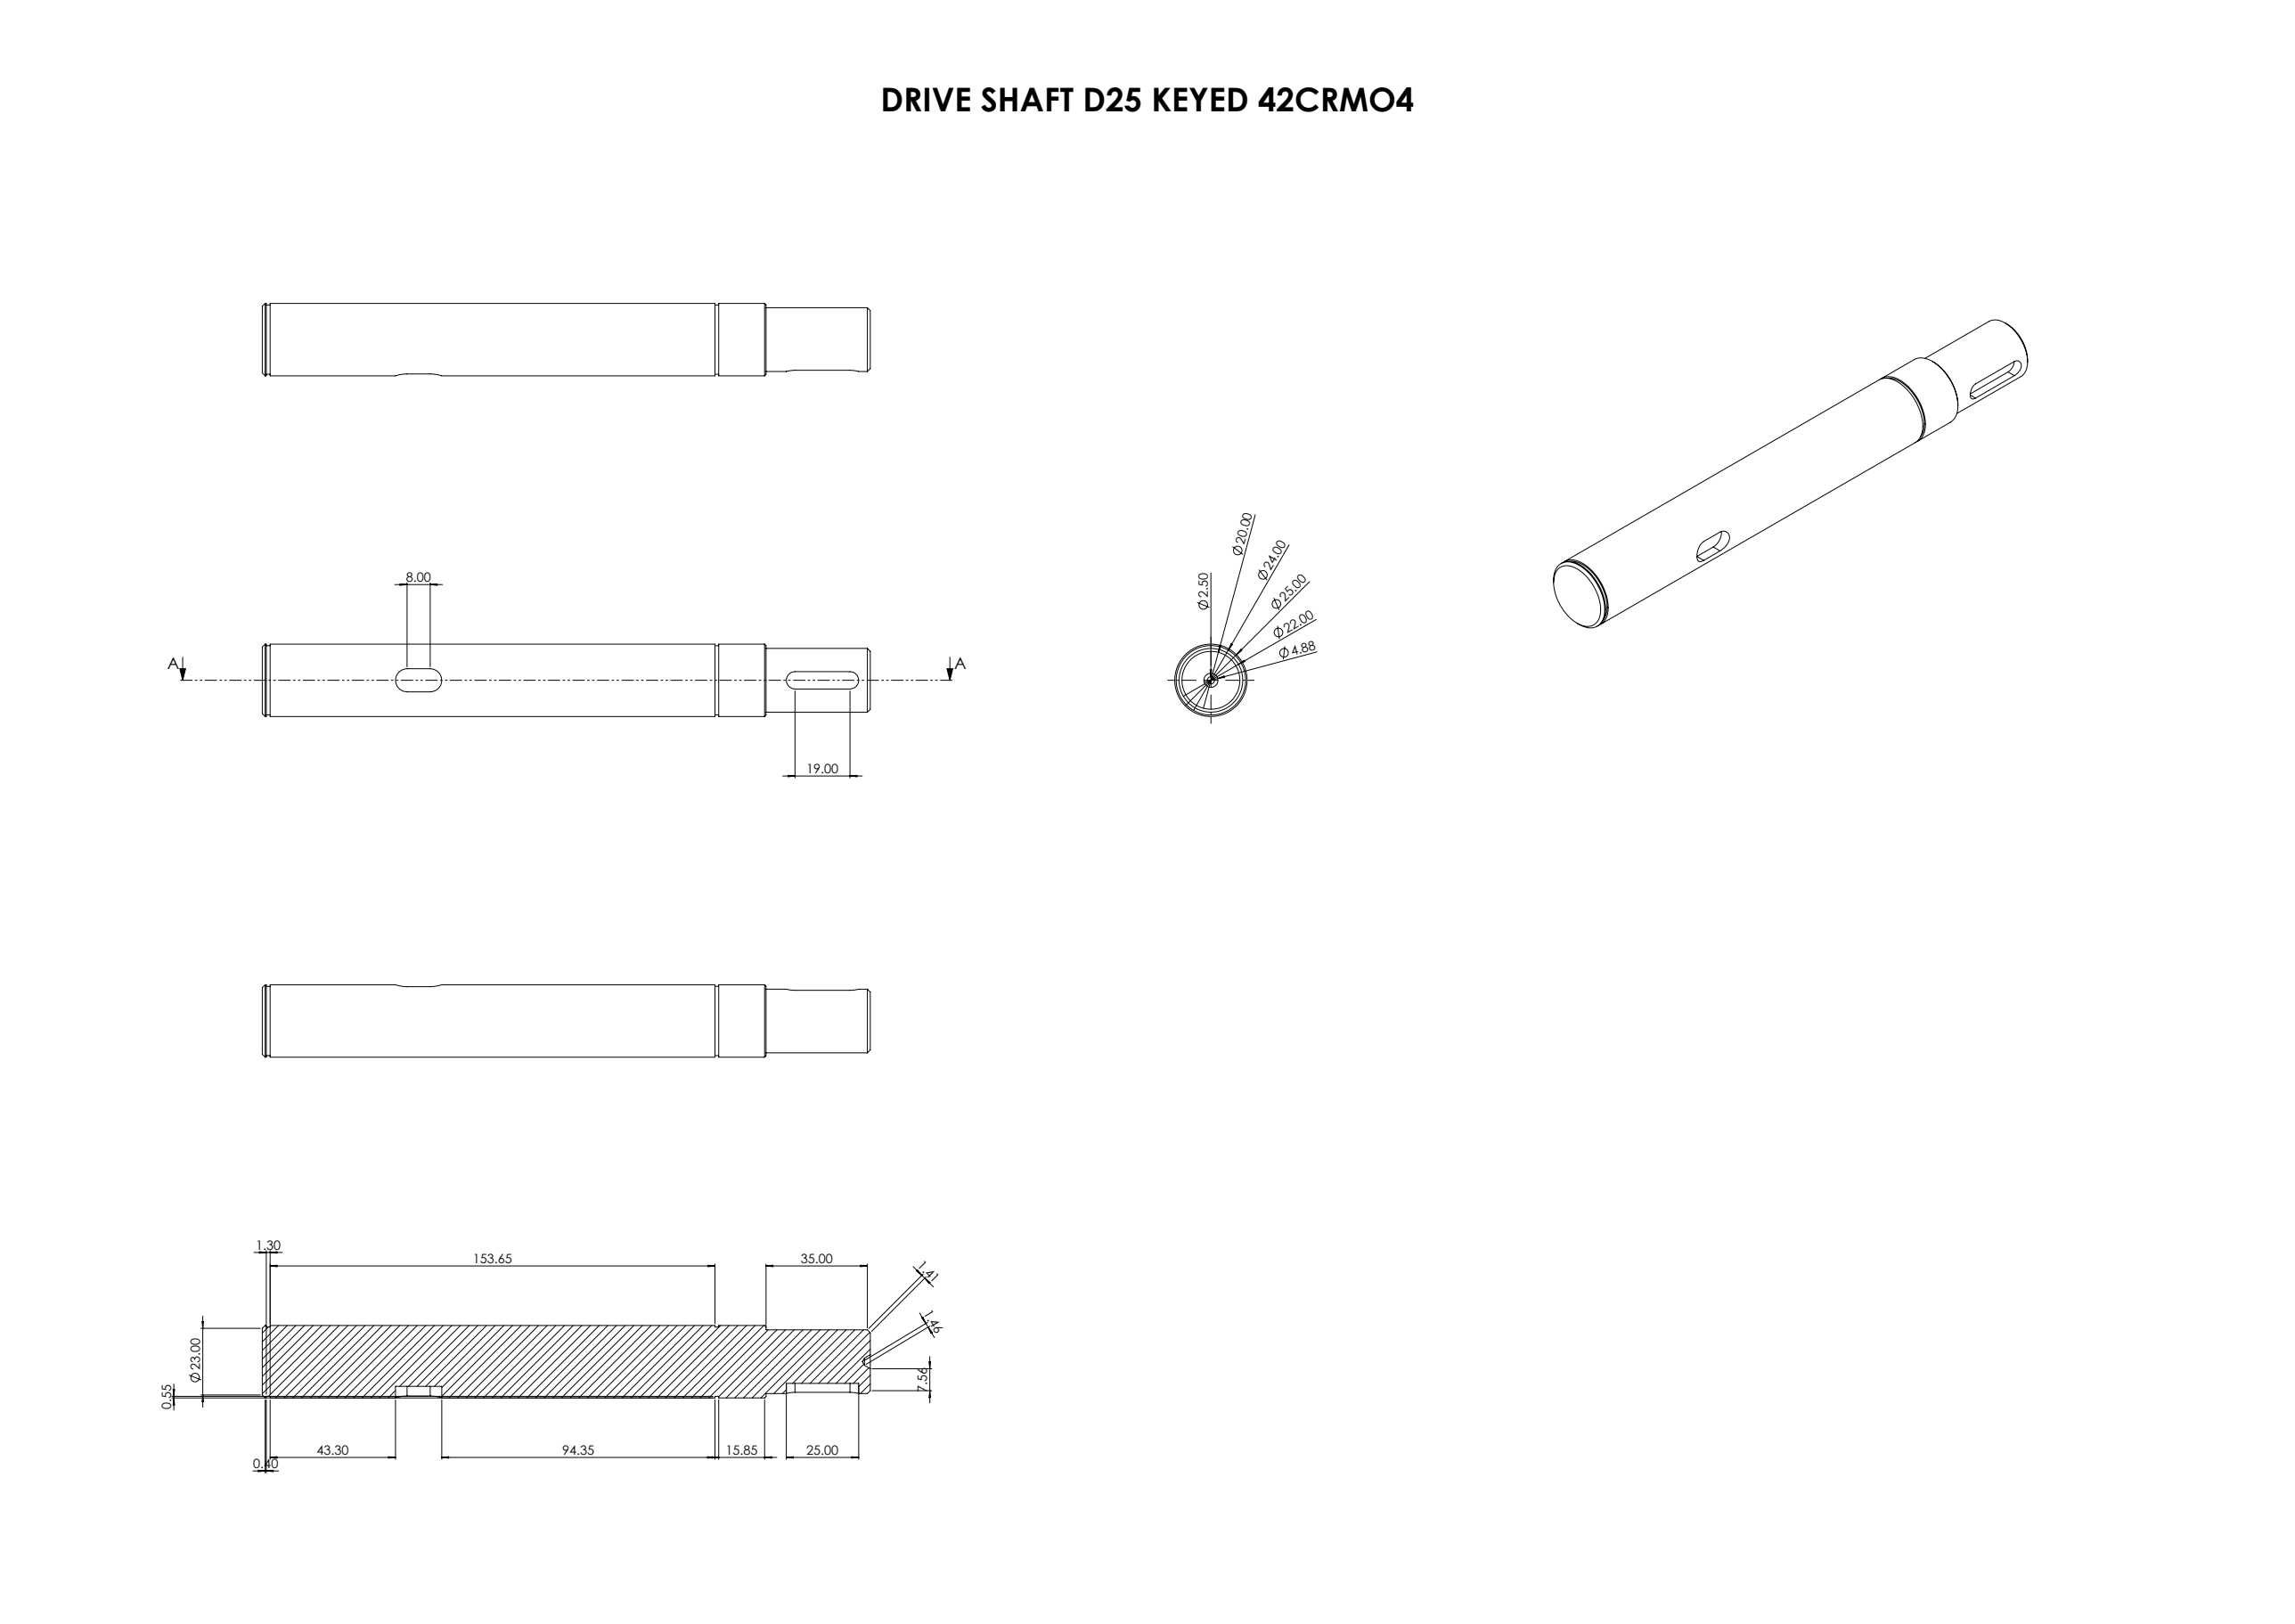
ISO-10303-21;
HEADER;
/* Generated by software containing ST-Developer
 * from STEP Tools, Inc. (www.steptools.com) 
 */

FILE_DESCRIPTION(
/* description */ (''),
/* implementation_level */ '2;1');

FILE_NAME(
/* name */ '04_Drive_Shaft_D25_Keyed_42CrMo4.step',
/* time_stamp */ '2026-10-23T00:52:27+05:00',
/* author */ (''),
/* organization */ (''),
/* preprocessor_version */ 'ST-DEVELOPER v20.2',
/* originating_system */ 'Autodesk Translation Framework v15.15.0.0',
/* authorisation */ '');

FILE_SCHEMA (('AUTOMOTIVE_DESIGN { 1 0 10303 214 3 1 1 }'));
ENDSEC;

DATA;
#10=MECHANICAL_DESIGN_GEOMETRIC_PRESENTATION_REPRESENTATION('',(#1556),#59204);
#679=B_SPLINE_CURVE_WITH_KNOTS('',3,(#41868,#41869,#41870,#41871,#41872,
#41873,#41874,#41875,#41876,#41877,#41878,#41879,#41880,#41881,#41882,#41883,
#41884,#41885),.UNSPECIFIED.,.F.,.F.,(4,2,2,2,2,2,2,2,4),(-0.909033920514541,
-0.795393296746547,-0.681752672978553,-0.568134816617911,-0.45451696025727,
-0.340899103896629,-0.227281247535988,-0.113640623767994,0.),
 .UNSPECIFIED.);
#680=B_SPLINE_CURVE_WITH_KNOTS('',3,(#41896,#41897,#41898,#41899,#41900,
#41901,#41902,#41903,#41904,#41905,#41906,#41907,#41908,#41909,#41910,#41911,
#41912,#41913),.UNSPECIFIED.,.F.,.F.,(4,2,2,2,2,2,2,2,4),(0.,0.113640623767995,
0.22728124753599,0.34089910389663,0.454516960257271,0.568134816617911,0.681752672978552,
0.795393296746547,0.909033920514541),.UNSPECIFIED.);
#681=B_SPLINE_CURVE_WITH_KNOTS('',3,(#41927,#41928,#41929,#41930,#41931,
#41932,#41933,#41934,#41935,#41936,#41937,#41938,#41939,#41940,#41941,#41942,
#41943,#41944),.UNSPECIFIED.,.F.,.F.,(4,2,2,2,2,2,2,2,4),(-1.21468374386295,
-1.06281862619298,-0.910953508522999,-0.759147690227238,-0.607341871931477,
-0.455536053635716,-0.303730235339955,-0.151865117669978,0.),
 .UNSPECIFIED.);
#682=B_SPLINE_CURVE_WITH_KNOTS('',3,(#41955,#41956,#41957,#41958,#41959,
#41960,#41961,#41962,#41963,#41964,#41965,#41966,#41967,#41968,#41969,#41970,
#41971,#41972),.UNSPECIFIED.,.F.,.F.,(4,2,2,2,2,2,2,2,4),(0.,0.151865117669977,
0.303730235339955,0.455536053635716,0.607341871931477,0.759147690227237,
0.910953508522998,1.06281862619298,1.21468374386295),.UNSPECIFIED.);
#1516=SHAPE_REPRESENTATION_RELATIONSHIP('SRR','None',#59305,#1536);
#1536=ADVANCED_BREP_SHAPE_REPRESENTATION('',(#1583),#59192);
#1556=STYLED_ITEM('',(#59586),#1583);
#1583=MANIFOLD_SOLID_BREP('Drive shaft',#22812);
#1639=FACE_BOUND('',#4332,.T.);
#1640=FACE_BOUND('',#4335,.T.);
#1641=FACE_BOUND('',#4337,.T.);
#1642=FACE_BOUND('',#4341,.T.);
#1643=FACE_BOUND('',#4344,.T.);
#1644=FACE_BOUND('',#4346,.T.);
#1645=FACE_BOUND('',#4348,.T.);
#1646=FACE_BOUND('',#4351,.T.);
#1990=PLANE('',#23564);
#1991=PLANE('',#23567);
#1992=PLANE('',#23570);
#1993=PLANE('',#23571);
#1994=PLANE('',#23574);
#1995=PLANE('',#23577);
#1996=PLANE('',#23578);
#1997=PLANE('',#23584);
#1998=PLANE('',#23590);
#1999=PLANE('',#23594);
#2000=PLANE('',#23598);
#2001=PLANE('',#23602);
#2002=PLANE('',#23608);
#2471=CYLINDRICAL_SURFACE('',#23565,0.3);
#2472=CYLINDRICAL_SURFACE('',#23568,0.3);
#2473=CYLINDRICAL_SURFACE('',#23572,0.4);
#2474=CYLINDRICAL_SURFACE('',#23575,0.4);
#2475=CYLINDRICAL_SURFACE('',#23582,1.1);
#2476=CYLINDRICAL_SURFACE('',#23588,1.25);
#2477=CYLINDRICAL_SURFACE('',#23592,1.195);
#2478=CYLINDRICAL_SURFACE('',#23596,1.25);
#2479=CYLINDRICAL_SURFACE('',#23600,1.195);
#2480=CYLINDRICAL_SURFACE('',#23604,1.25);
#2974=FACE_OUTER_BOUND('',#4319,.T.);
#2975=FACE_OUTER_BOUND('',#4320,.T.);
#2976=FACE_OUTER_BOUND('',#4321,.T.);
#2977=FACE_OUTER_BOUND('',#4322,.T.);
#2978=FACE_OUTER_BOUND('',#4323,.T.);
#2979=FACE_OUTER_BOUND('',#4324,.T.);
#2980=FACE_OUTER_BOUND('',#4325,.T.);
#2981=FACE_OUTER_BOUND('',#4326,.T.);
#2982=FACE_OUTER_BOUND('',#4327,.T.);
#2983=FACE_OUTER_BOUND('',#4328,.T.);
#2984=FACE_OUTER_BOUND('',#4329,.T.);
#2985=FACE_OUTER_BOUND('',#4330,.T.);
#2986=FACE_OUTER_BOUND('',#4331,.T.);
#2987=FACE_OUTER_BOUND('',#4333,.T.);
#2988=FACE_OUTER_BOUND('',#4334,.T.);
#2989=FACE_OUTER_BOUND('',#4336,.T.);
#2990=FACE_OUTER_BOUND('',#4338,.T.);
#2991=FACE_OUTER_BOUND('',#4339,.T.);
#2992=FACE_OUTER_BOUND('',#4340,.T.);
#2993=FACE_OUTER_BOUND('',#4342,.T.);
#2994=FACE_OUTER_BOUND('',#4343,.T.);
#2995=FACE_OUTER_BOUND('',#4345,.T.);
#2996=FACE_OUTER_BOUND('',#4347,.T.);
#2997=FACE_OUTER_BOUND('',#4349,.T.);
#2998=FACE_OUTER_BOUND('',#4350,.T.);
#2999=FACE_OUTER_BOUND('',#4352,.T.);
#3000=FACE_OUTER_BOUND('',#4353,.T.);
#3001=FACE_OUTER_BOUND('',#4354,.T.);
#4319=EDGE_LOOP('',(#16112,#16113,#16114,#16115));
#4320=EDGE_LOOP('',(#16116,#16117,#16118));
#4321=EDGE_LOOP('',(#16119,#16120,#16121,#16122));
#4322=EDGE_LOOP('',(#16123,#16124,#16125,#16126));
#4323=EDGE_LOOP('',(#16127,#16128,#16129,#16130));
#4324=EDGE_LOOP('',(#16131,#16132,#16133,#16134));
#4325=EDGE_LOOP('',(#16135,#16136,#16137,#16138));
#4326=EDGE_LOOP('',(#16139,#16140,#16141,#16142));
#4327=EDGE_LOOP('',(#16143,#16144,#16145,#16146));
#4328=EDGE_LOOP('',(#16147,#16148,#16149,#16150));
#4329=EDGE_LOOP('',(#16151,#16152,#16153,#16154));
#4330=EDGE_LOOP('',(#16155,#16156,#16157,#16158));
#4331=EDGE_LOOP('',(#16159));
#4332=EDGE_LOOP('',(#16160));
#4333=EDGE_LOOP('',(#16161,#16162,#16163,#16164));
#4334=EDGE_LOOP('',(#16165,#16166,#16167,#16168));
#4335=EDGE_LOOP('',(#16169,#16170,#16171,#16172));
#4336=EDGE_LOOP('',(#16173));
#4337=EDGE_LOOP('',(#16174));
#4338=EDGE_LOOP('',(#16175,#16176,#16177,#16178));
#4339=EDGE_LOOP('',(#16179,#16180,#16181,#16182));
#4340=EDGE_LOOP('',(#16183));
#4341=EDGE_LOOP('',(#16184));
#4342=EDGE_LOOP('',(#16185,#16186,#16187,#16188));
#4343=EDGE_LOOP('',(#16189));
#4344=EDGE_LOOP('',(#16190));
#4345=EDGE_LOOP('',(#16191,#16192,#16193,#16194));
#4346=EDGE_LOOP('',(#16195,#16196,#16197,#16198));
#4347=EDGE_LOOP('',(#16199));
#4348=EDGE_LOOP('',(#16200));
#4349=EDGE_LOOP('',(#16201,#16202,#16203,#16204));
#4350=EDGE_LOOP('',(#16205));
#4351=EDGE_LOOP('',(#16206));
#4352=EDGE_LOOP('',(#16207,#16208,#16209,#16210));
#4353=EDGE_LOOP('',(#16211,#16212,#16213,#16214));
#4354=EDGE_LOOP('',(#16215));
#5857=LINE('',#41852,#7290);
#5858=LINE('',#41856,#7291);
#5859=LINE('',#41860,#7292);
#5860=LINE('',#41862,#7293);
#5861=LINE('',#41864,#7294);
#5862=LINE('',#41865,#7295);
#5863=LINE('',#41888,#7296);
#5864=LINE('',#41891,#7297);
#5865=LINE('',#41893,#7298);
#5866=LINE('',#41894,#7299);
#5867=LINE('',#41919,#7300);
#5868=LINE('',#41921,#7301);
#5869=LINE('',#41923,#7302);
#5870=LINE('',#41924,#7303);
#5871=LINE('',#41947,#7304);
#5872=LINE('',#41950,#7305);
#5873=LINE('',#41952,#7306);
#5874=LINE('',#41953,#7307);
#5875=LINE('',#41981,#7308);
#5876=LINE('',#41985,#7309);
#5877=LINE('',#41992,#7310);
#5878=LINE('',#41996,#7311);
#5879=LINE('',#42003,#7312);
#5880=LINE('',#42010,#7313);
#5881=LINE('',#42017,#7314);
#5882=LINE('',#42024,#7315);
#5883=LINE('',#42028,#7316);
#7290=VECTOR('',#26517,0.1875);
#7291=VECTOR('',#26522,0.125);
#7292=VECTOR('',#26525,1.);
#7293=VECTOR('',#26526,1.);
#7294=VECTOR('',#26527,1.);
#7295=VECTOR('',#26528,1.);
#7296=VECTOR('',#26533,1.);
#7297=VECTOR('',#26536,1.);
#7298=VECTOR('',#26537,1.);
#7299=VECTOR('',#26538,1.);
#7300=VECTOR('',#26547,1.);
#7301=VECTOR('',#26548,1.);
#7302=VECTOR('',#26549,1.);
#7303=VECTOR('',#26550,1.);
#7304=VECTOR('',#26555,1.);
#7305=VECTOR('',#26558,1.);
#7306=VECTOR('',#26559,1.);
#7307=VECTOR('',#26560,1.);
#7308=VECTOR('',#26575,1.05);
#7309=VECTOR('',#26580,1.1);
#7310=VECTOR('',#26589,1.225);
#7311=VECTOR('',#26594,1.25);
#7312=VECTOR('',#26603,1.195);
#7313=VECTOR('',#26612,1.25);
#7314=VECTOR('',#26621,1.195);
#7315=VECTOR('',#26630,1.25);
#7316=VECTOR('',#26635,1.2);
#8574=CIRCLE('',#23561,0.24404761904762);
#8575=CIRCLE('',#23562,0.125);
#8576=CIRCLE('',#23566,0.3);
#8577=CIRCLE('',#23569,0.3);
#8578=CIRCLE('',#23573,0.4);
#8579=CIRCLE('',#23576,0.4);
#8580=CIRCLE('',#23579,1.);
#8581=CIRCLE('',#23581,1.1);
#8582=CIRCLE('',#23583,1.1);
#8583=CIRCLE('',#23585,1.2);
#8584=CIRCLE('',#23587,1.25);
#8585=CIRCLE('',#23589,1.25);
#8586=CIRCLE('',#23591,1.195);
#8587=CIRCLE('',#23593,1.195);
#8588=CIRCLE('',#23595,1.25);
#8589=CIRCLE('',#23597,1.25);
#8590=CIRCLE('',#23599,1.195);
#8591=CIRCLE('',#23601,1.195);
#8592=CIRCLE('',#23603,1.25);
#8593=CIRCLE('',#23605,1.25);
#8594=CIRCLE('',#23607,1.15);
#9642=VERTEX_POINT('',#41849);
#9643=VERTEX_POINT('',#41851);
#9644=VERTEX_POINT('',#41855);
#9645=VERTEX_POINT('',#41858);
#9646=VERTEX_POINT('',#41859);
#9647=VERTEX_POINT('',#41861);
#9648=VERTEX_POINT('',#41863);
#9649=VERTEX_POINT('',#41867);
#9650=VERTEX_POINT('',#41886);
#9651=VERTEX_POINT('',#41890);
#9652=VERTEX_POINT('',#41892);
#9653=VERTEX_POINT('',#41917);
#9654=VERTEX_POINT('',#41918);
#9655=VERTEX_POINT('',#41920);
#9656=VERTEX_POINT('',#41922);
#9657=VERTEX_POINT('',#41926);
#9658=VERTEX_POINT('',#41945);
#9659=VERTEX_POINT('',#41949);
#9660=VERTEX_POINT('',#41951);
#9661=VERTEX_POINT('',#41976);
#9662=VERTEX_POINT('',#41979);
#9663=VERTEX_POINT('',#41983);
#9664=VERTEX_POINT('',#41987);
#9665=VERTEX_POINT('',#41990);
#9666=VERTEX_POINT('',#41994);
#9667=VERTEX_POINT('',#41998);
#9668=VERTEX_POINT('',#42001);
#9669=VERTEX_POINT('',#42005);
#9670=VERTEX_POINT('',#42008);
#9671=VERTEX_POINT('',#42012);
#9672=VERTEX_POINT('',#42015);
#9673=VERTEX_POINT('',#42019);
#9674=VERTEX_POINT('',#42022);
#9675=VERTEX_POINT('',#42026);
#12060=EDGE_CURVE('',#9642,#9642,#8574,.T.);
#12061=EDGE_CURVE('',#9642,#9643,#5857,.T.);
#12062=EDGE_CURVE('',#9643,#9643,#8575,.T.);
#12063=EDGE_CURVE('',#9643,#9644,#5858,.T.);
#12064=EDGE_CURVE('',#9645,#9646,#5859,.T.);
#12065=EDGE_CURVE('',#9647,#9645,#5860,.T.);
#12066=EDGE_CURVE('',#9647,#9648,#5861,.T.);
#12067=EDGE_CURVE('',#9648,#9646,#5862,.T.);
#12068=EDGE_CURVE('',#9646,#9649,#679,.T.);
#12069=EDGE_CURVE('',#9650,#9648,#8576,.T.);
#12070=EDGE_CURVE('',#9650,#9649,#5863,.T.);
#12071=EDGE_CURVE('',#9649,#9651,#5864,.T.);
#12072=EDGE_CURVE('',#9650,#9652,#5865,.T.);
#12073=EDGE_CURVE('',#9652,#9651,#5866,.T.);
#12074=EDGE_CURVE('',#9651,#9645,#680,.T.);
#12075=EDGE_CURVE('',#9647,#9652,#8577,.T.);
#12076=EDGE_CURVE('',#9653,#9654,#5867,.T.);
#12077=EDGE_CURVE('',#9655,#9653,#5868,.T.);
#12078=EDGE_CURVE('',#9655,#9656,#5869,.T.);
#12079=EDGE_CURVE('',#9656,#9654,#5870,.T.);
#12080=EDGE_CURVE('',#9654,#9657,#681,.T.);
#12081=EDGE_CURVE('',#9658,#9656,#8578,.T.);
#12082=EDGE_CURVE('',#9658,#9657,#5871,.T.);
#12083=EDGE_CURVE('',#9657,#9659,#5872,.T.);
#12084=EDGE_CURVE('',#9658,#9660,#5873,.T.);
#12085=EDGE_CURVE('',#9660,#9659,#5874,.T.);
#12086=EDGE_CURVE('',#9659,#9653,#682,.T.);
#12087=EDGE_CURVE('',#9655,#9660,#8579,.T.);
#12088=EDGE_CURVE('',#9661,#9661,#8580,.T.);
#12089=EDGE_CURVE('',#9662,#9662,#8581,.T.);
#12090=EDGE_CURVE('',#9662,#9661,#5875,.T.);
#12091=EDGE_CURVE('',#9663,#9663,#8582,.T.);
#12092=EDGE_CURVE('',#9663,#9662,#5876,.T.);
#12093=EDGE_CURVE('',#9664,#9664,#8583,.T.);
#12094=EDGE_CURVE('',#9665,#9665,#8584,.T.);
#12095=EDGE_CURVE('',#9665,#9664,#5877,.T.);
#12096=EDGE_CURVE('',#9666,#9666,#8585,.T.);
#12097=EDGE_CURVE('',#9666,#9665,#5878,.T.);
#12098=EDGE_CURVE('',#9667,#9667,#8586,.T.);
#12099=EDGE_CURVE('',#9668,#9668,#8587,.T.);
#12100=EDGE_CURVE('',#9668,#9667,#5879,.T.);
#12101=EDGE_CURVE('',#9669,#9669,#8588,.T.);
#12102=EDGE_CURVE('',#9670,#9670,#8589,.T.);
#12103=EDGE_CURVE('',#9670,#9669,#5880,.T.);
#12104=EDGE_CURVE('',#9671,#9671,#8590,.T.);
#12105=EDGE_CURVE('',#9672,#9672,#8591,.T.);
#12106=EDGE_CURVE('',#9672,#9671,#5881,.T.);
#12107=EDGE_CURVE('',#9673,#9673,#8592,.T.);
#12108=EDGE_CURVE('',#9674,#9674,#8593,.T.);
#12109=EDGE_CURVE('',#9674,#9673,#5882,.T.);
#12110=EDGE_CURVE('',#9675,#9675,#8594,.T.);
#12111=EDGE_CURVE('',#9675,#9674,#5883,.T.);
#16112=ORIENTED_EDGE('',*,*,#12060,.F.);
#16113=ORIENTED_EDGE('',*,*,#12061,.T.);
#16114=ORIENTED_EDGE('',*,*,#12062,.T.);
#16115=ORIENTED_EDGE('',*,*,#12061,.F.);
#16116=ORIENTED_EDGE('',*,*,#12062,.F.);
#16117=ORIENTED_EDGE('',*,*,#12063,.T.);
#16118=ORIENTED_EDGE('',*,*,#12063,.F.);
#16119=ORIENTED_EDGE('',*,*,#12064,.F.);
#16120=ORIENTED_EDGE('',*,*,#12065,.F.);
#16121=ORIENTED_EDGE('',*,*,#12066,.T.);
#16122=ORIENTED_EDGE('',*,*,#12067,.T.);
#16123=ORIENTED_EDGE('',*,*,#12068,.F.);
#16124=ORIENTED_EDGE('',*,*,#12067,.F.);
#16125=ORIENTED_EDGE('',*,*,#12069,.F.);
#16126=ORIENTED_EDGE('',*,*,#12070,.T.);
#16127=ORIENTED_EDGE('',*,*,#12071,.F.);
#16128=ORIENTED_EDGE('',*,*,#12070,.F.);
#16129=ORIENTED_EDGE('',*,*,#12072,.T.);
#16130=ORIENTED_EDGE('',*,*,#12073,.T.);
#16131=ORIENTED_EDGE('',*,*,#12074,.F.);
#16132=ORIENTED_EDGE('',*,*,#12073,.F.);
#16133=ORIENTED_EDGE('',*,*,#12075,.F.);
#16134=ORIENTED_EDGE('',*,*,#12065,.T.);
#16135=ORIENTED_EDGE('',*,*,#12069,.T.);
#16136=ORIENTED_EDGE('',*,*,#12066,.F.);
#16137=ORIENTED_EDGE('',*,*,#12075,.T.);
#16138=ORIENTED_EDGE('',*,*,#12072,.F.);
#16139=ORIENTED_EDGE('',*,*,#12076,.F.);
#16140=ORIENTED_EDGE('',*,*,#12077,.F.);
#16141=ORIENTED_EDGE('',*,*,#12078,.T.);
#16142=ORIENTED_EDGE('',*,*,#12079,.T.);
#16143=ORIENTED_EDGE('',*,*,#12080,.F.);
#16144=ORIENTED_EDGE('',*,*,#12079,.F.);
#16145=ORIENTED_EDGE('',*,*,#12081,.F.);
#16146=ORIENTED_EDGE('',*,*,#12082,.T.);
#16147=ORIENTED_EDGE('',*,*,#12083,.F.);
#16148=ORIENTED_EDGE('',*,*,#12082,.F.);
#16149=ORIENTED_EDGE('',*,*,#12084,.T.);
#16150=ORIENTED_EDGE('',*,*,#12085,.T.);
#16151=ORIENTED_EDGE('',*,*,#12086,.F.);
#16152=ORIENTED_EDGE('',*,*,#12085,.F.);
#16153=ORIENTED_EDGE('',*,*,#12087,.F.);
#16154=ORIENTED_EDGE('',*,*,#12077,.T.);
#16155=ORIENTED_EDGE('',*,*,#12081,.T.);
#16156=ORIENTED_EDGE('',*,*,#12078,.F.);
#16157=ORIENTED_EDGE('',*,*,#12087,.T.);
#16158=ORIENTED_EDGE('',*,*,#12084,.F.);
#16159=ORIENTED_EDGE('',*,*,#12088,.F.);
#16160=ORIENTED_EDGE('',*,*,#12060,.T.);
#16161=ORIENTED_EDGE('',*,*,#12089,.F.);
#16162=ORIENTED_EDGE('',*,*,#12090,.T.);
#16163=ORIENTED_EDGE('',*,*,#12088,.T.);
#16164=ORIENTED_EDGE('',*,*,#12090,.F.);
#16165=ORIENTED_EDGE('',*,*,#12091,.F.);
#16166=ORIENTED_EDGE('',*,*,#12092,.T.);
#16167=ORIENTED_EDGE('',*,*,#12089,.T.);
#16168=ORIENTED_EDGE('',*,*,#12092,.F.);
#16169=ORIENTED_EDGE('',*,*,#12071,.T.);
#16170=ORIENTED_EDGE('',*,*,#12074,.T.);
#16171=ORIENTED_EDGE('',*,*,#12064,.T.);
#16172=ORIENTED_EDGE('',*,*,#12068,.T.);
#16173=ORIENTED_EDGE('',*,*,#12093,.F.);
#16174=ORIENTED_EDGE('',*,*,#12091,.T.);
#16175=ORIENTED_EDGE('',*,*,#12094,.F.);
#16176=ORIENTED_EDGE('',*,*,#12095,.T.);
#16177=ORIENTED_EDGE('',*,*,#12093,.T.);
#16178=ORIENTED_EDGE('',*,*,#12095,.F.);
#16179=ORIENTED_EDGE('',*,*,#12096,.F.);
#16180=ORIENTED_EDGE('',*,*,#12097,.T.);
#16181=ORIENTED_EDGE('',*,*,#12094,.T.);
#16182=ORIENTED_EDGE('',*,*,#12097,.F.);
#16183=ORIENTED_EDGE('',*,*,#12096,.T.);
#16184=ORIENTED_EDGE('',*,*,#12098,.F.);
#16185=ORIENTED_EDGE('',*,*,#12099,.F.);
#16186=ORIENTED_EDGE('',*,*,#12100,.T.);
#16187=ORIENTED_EDGE('',*,*,#12098,.T.);
#16188=ORIENTED_EDGE('',*,*,#12100,.F.);
#16189=ORIENTED_EDGE('',*,*,#12101,.F.);
#16190=ORIENTED_EDGE('',*,*,#12099,.T.);
#16191=ORIENTED_EDGE('',*,*,#12102,.F.);
#16192=ORIENTED_EDGE('',*,*,#12103,.T.);
#16193=ORIENTED_EDGE('',*,*,#12101,.T.);
#16194=ORIENTED_EDGE('',*,*,#12103,.F.);
#16195=ORIENTED_EDGE('',*,*,#12083,.T.);
#16196=ORIENTED_EDGE('',*,*,#12086,.T.);
#16197=ORIENTED_EDGE('',*,*,#12076,.T.);
#16198=ORIENTED_EDGE('',*,*,#12080,.T.);
#16199=ORIENTED_EDGE('',*,*,#12102,.T.);
#16200=ORIENTED_EDGE('',*,*,#12104,.F.);
#16201=ORIENTED_EDGE('',*,*,#12105,.F.);
#16202=ORIENTED_EDGE('',*,*,#12106,.T.);
#16203=ORIENTED_EDGE('',*,*,#12104,.T.);
#16204=ORIENTED_EDGE('',*,*,#12106,.F.);
#16205=ORIENTED_EDGE('',*,*,#12107,.F.);
#16206=ORIENTED_EDGE('',*,*,#12105,.T.);
#16207=ORIENTED_EDGE('',*,*,#12108,.F.);
#16208=ORIENTED_EDGE('',*,*,#12109,.T.);
#16209=ORIENTED_EDGE('',*,*,#12107,.T.);
#16210=ORIENTED_EDGE('',*,*,#12109,.F.);
#16211=ORIENTED_EDGE('',*,*,#12110,.F.);
#16212=ORIENTED_EDGE('',*,*,#12111,.T.);
#16213=ORIENTED_EDGE('',*,*,#12108,.T.);
#16214=ORIENTED_EDGE('',*,*,#12111,.F.);
#16215=ORIENTED_EDGE('',*,*,#12110,.T.);
#21359=CONICAL_SURFACE('',#23560,0.1875,0.536910742740044);
#21360=CONICAL_SURFACE('',#23563,0.125,1.03037682652432);
#21361=CONICAL_SURFACE('',#23580,1.05,0.785398163397442);
#21362=CONICAL_SURFACE('',#23586,1.225,0.785398163397442);
#21363=CONICAL_SURFACE('',#23606,1.2,0.785398163397446);
#21804=ADVANCED_FACE('',(#2974),#21359,.F.);
#21805=ADVANCED_FACE('',(#2975),#21360,.F.);
#21806=ADVANCED_FACE('',(#2976),#1990,.F.);
#21807=ADVANCED_FACE('',(#2977),#2471,.F.);
#21808=ADVANCED_FACE('',(#2978),#1991,.F.);
#21809=ADVANCED_FACE('',(#2979),#2472,.F.);
#21810=ADVANCED_FACE('',(#2980),#1992,.T.);
#21811=ADVANCED_FACE('',(#2981),#1993,.F.);
#21812=ADVANCED_FACE('',(#2982),#2473,.F.);
#21813=ADVANCED_FACE('',(#2983),#1994,.F.);
#21814=ADVANCED_FACE('',(#2984),#2474,.F.);
#21815=ADVANCED_FACE('',(#2985),#1995,.T.);
#21816=ADVANCED_FACE('',(#2986,#1639),#1996,.T.);
#21817=ADVANCED_FACE('',(#2987),#21361,.T.);
#21818=ADVANCED_FACE('',(#2988,#1640),#2475,.T.);
#21819=ADVANCED_FACE('',(#2989,#1641),#1997,.T.);
#21820=ADVANCED_FACE('',(#2990),#21362,.T.);
#21821=ADVANCED_FACE('',(#2991),#2476,.T.);
#21822=ADVANCED_FACE('',(#2992,#1642),#1998,.T.);
#21823=ADVANCED_FACE('',(#2993),#2477,.T.);
#21824=ADVANCED_FACE('',(#2994,#1643),#1999,.T.);
#21825=ADVANCED_FACE('',(#2995,#1644),#2478,.T.);
#21826=ADVANCED_FACE('',(#2996,#1645),#2000,.T.);
#21827=ADVANCED_FACE('',(#2997),#2479,.T.);
#21828=ADVANCED_FACE('',(#2998,#1646),#2001,.T.);
#21829=ADVANCED_FACE('',(#2999),#2480,.T.);
#21830=ADVANCED_FACE('',(#3000),#21363,.T.);
#21831=ADVANCED_FACE('',(#3001),#2002,.T.);
#22812=CLOSED_SHELL('',(#21804,#21805,#21806,#21807,#21808,#21809,#21810,
#21811,#21812,#21813,#21814,#21815,#21816,#21817,#21818,#21819,#21820,#21821,
#21822,#21823,#21824,#21825,#21826,#21827,#21828,#21829,#21830,#21831));
#23559=AXIS2_PLACEMENT_3D('',#41847,#26511,#26512);
#23560=AXIS2_PLACEMENT_3D('',#41848,#26513,#26514);
#23561=AXIS2_PLACEMENT_3D('',#41850,#26515,#26516);
#23562=AXIS2_PLACEMENT_3D('',#41853,#26518,#26519);
#23563=AXIS2_PLACEMENT_3D('',#41854,#26520,#26521);
#23564=AXIS2_PLACEMENT_3D('',#41857,#26523,#26524);
#23565=AXIS2_PLACEMENT_3D('',#41866,#26529,#26530);
#23566=AXIS2_PLACEMENT_3D('',#41887,#26531,#26532);
#23567=AXIS2_PLACEMENT_3D('',#41889,#26534,#26535);
#23568=AXIS2_PLACEMENT_3D('',#41895,#26539,#26540);
#23569=AXIS2_PLACEMENT_3D('',#41914,#26541,#26542);
#23570=AXIS2_PLACEMENT_3D('',#41915,#26543,#26544);
#23571=AXIS2_PLACEMENT_3D('',#41916,#26545,#26546);
#23572=AXIS2_PLACEMENT_3D('',#41925,#26551,#26552);
#23573=AXIS2_PLACEMENT_3D('',#41946,#26553,#26554);
#23574=AXIS2_PLACEMENT_3D('',#41948,#26556,#26557);
#23575=AXIS2_PLACEMENT_3D('',#41954,#26561,#26562);
#23576=AXIS2_PLACEMENT_3D('',#41973,#26563,#26564);
#23577=AXIS2_PLACEMENT_3D('',#41974,#26565,#26566);
#23578=AXIS2_PLACEMENT_3D('',#41975,#26567,#26568);
#23579=AXIS2_PLACEMENT_3D('',#41977,#26569,#26570);
#23580=AXIS2_PLACEMENT_3D('',#41978,#26571,#26572);
#23581=AXIS2_PLACEMENT_3D('',#41980,#26573,#26574);
#23582=AXIS2_PLACEMENT_3D('',#41982,#26576,#26577);
#23583=AXIS2_PLACEMENT_3D('',#41984,#26578,#26579);
#23584=AXIS2_PLACEMENT_3D('',#41986,#26581,#26582);
#23585=AXIS2_PLACEMENT_3D('',#41988,#26583,#26584);
#23586=AXIS2_PLACEMENT_3D('',#41989,#26585,#26586);
#23587=AXIS2_PLACEMENT_3D('',#41991,#26587,#26588);
#23588=AXIS2_PLACEMENT_3D('',#41993,#26590,#26591);
#23589=AXIS2_PLACEMENT_3D('',#41995,#26592,#26593);
#23590=AXIS2_PLACEMENT_3D('',#41997,#26595,#26596);
#23591=AXIS2_PLACEMENT_3D('',#41999,#26597,#26598);
#23592=AXIS2_PLACEMENT_3D('',#42000,#26599,#26600);
#23593=AXIS2_PLACEMENT_3D('',#42002,#26601,#26602);
#23594=AXIS2_PLACEMENT_3D('',#42004,#26604,#26605);
#23595=AXIS2_PLACEMENT_3D('',#42006,#26606,#26607);
#23596=AXIS2_PLACEMENT_3D('',#42007,#26608,#26609);
#23597=AXIS2_PLACEMENT_3D('',#42009,#26610,#26611);
#23598=AXIS2_PLACEMENT_3D('',#42011,#26613,#26614);
#23599=AXIS2_PLACEMENT_3D('',#42013,#26615,#26616);
#23600=AXIS2_PLACEMENT_3D('',#42014,#26617,#26618);
#23601=AXIS2_PLACEMENT_3D('',#42016,#26619,#26620);
#23602=AXIS2_PLACEMENT_3D('',#42018,#26622,#26623);
#23603=AXIS2_PLACEMENT_3D('',#42020,#26624,#26625);
#23604=AXIS2_PLACEMENT_3D('',#42021,#26626,#26627);
#23605=AXIS2_PLACEMENT_3D('',#42023,#26628,#26629);
#23606=AXIS2_PLACEMENT_3D('',#42025,#26631,#26632);
#23607=AXIS2_PLACEMENT_3D('',#42027,#26633,#26634);
#23608=AXIS2_PLACEMENT_3D('',#42029,#26636,#26637);
#26511=DIRECTION('axis',(0.,0.,1.));
#26512=DIRECTION('refdir',(1.,0.,0.));
#26513=DIRECTION('center_axis',(0.,0.,-1.));
#26514=DIRECTION('ref_axis',(1.,0.,0.));
#26515=DIRECTION('center_axis',(0.,0.,1.));
#26516=DIRECTION('ref_axis',(1.,0.,0.));
#26517=DIRECTION('',(0.511483859767681,6.26387071680024E-17,0.859292884409708));
#26518=DIRECTION('center_axis',(0.,0.,1.));
#26519=DIRECTION('ref_axis',(1.,0.,0.));
#26520=DIRECTION('center_axis',(0.,0.,-1.));
#26521=DIRECTION('ref_axis',(1.,0.,0.));
#26522=DIRECTION('',(0.857492925712546,1.05012596676537E-16,0.514495755427523));
#26523=DIRECTION('center_axis',(0.,-1.,0.));
#26524=DIRECTION('ref_axis',(0.,0.,-1.));
#26525=DIRECTION('',(0.,0.,1.));
#26526=DIRECTION('',(1.,0.,0.));
#26527=DIRECTION('',(0.,0.,1.));
#26528=DIRECTION('',(1.,0.,0.));
#26529=DIRECTION('center_axis',(1.,0.,0.));
#26530=DIRECTION('ref_axis',(0.,1.,0.));
#26531=DIRECTION('center_axis',(1.,0.,0.));
#26532=DIRECTION('ref_axis',(0.,1.,0.));
#26533=DIRECTION('',(1.,0.,0.));
#26534=DIRECTION('center_axis',(0.,1.,0.));
#26535=DIRECTION('ref_axis',(0.,0.,1.));
#26536=DIRECTION('',(0.,0.,-1.));
#26537=DIRECTION('',(0.,0.,-1.));
#26538=DIRECTION('',(1.,0.,0.));
#26539=DIRECTION('center_axis',(1.,0.,0.));
#26540=DIRECTION('ref_axis',(0.,-1.,0.));
#26541=DIRECTION('center_axis',(1.,0.,0.));
#26542=DIRECTION('ref_axis',(0.,-1.,0.));
#26543=DIRECTION('center_axis',(1.,0.,0.));
#26544=DIRECTION('ref_axis',(0.,0.,-1.));
#26545=DIRECTION('center_axis',(0.,-1.,0.));
#26546=DIRECTION('ref_axis',(0.,0.,-1.));
#26547=DIRECTION('',(0.,0.,1.));
#26548=DIRECTION('',(1.,0.,0.));
#26549=DIRECTION('',(0.,0.,1.));
#26550=DIRECTION('',(1.,0.,0.));
#26551=DIRECTION('center_axis',(1.,0.,0.));
#26552=DIRECTION('ref_axis',(0.,1.,2.77555756156289E-16));
#26553=DIRECTION('center_axis',(1.,0.,0.));
#26554=DIRECTION('ref_axis',(0.,1.,2.77555756156289E-16));
#26555=DIRECTION('',(1.,0.,0.));
#26556=DIRECTION('center_axis',(0.,1.,0.));
#26557=DIRECTION('ref_axis',(0.,0.,1.));
#26558=DIRECTION('',(0.,0.,-1.));
#26559=DIRECTION('',(0.,0.,-1.));
#26560=DIRECTION('',(1.,0.,0.));
#26561=DIRECTION('center_axis',(1.,0.,0.));
#26562=DIRECTION('ref_axis',(0.,-1.,5.55111512312578E-16));
#26563=DIRECTION('center_axis',(1.,0.,0.));
#26564=DIRECTION('ref_axis',(0.,-1.,5.55111512312578E-16));
#26565=DIRECTION('center_axis',(1.,0.,0.));
#26566=DIRECTION('ref_axis',(0.,0.,-1.));
#26567=DIRECTION('center_axis',(0.,0.,-1.));
#26568=DIRECTION('ref_axis',(-1.,0.,0.));
#26569=DIRECTION('center_axis',(0.,0.,1.));
#26570=DIRECTION('ref_axis',(1.,0.,0.));
#26571=DIRECTION('center_axis',(0.,0.,1.));
#26572=DIRECTION('ref_axis',(1.,0.,0.));
#26573=DIRECTION('center_axis',(0.,0.,1.));
#26574=DIRECTION('ref_axis',(1.,0.,0.));
#26575=DIRECTION('',(0.707106781186543,8.65956056235488E-17,-0.707106781186552));
#26576=DIRECTION('center_axis',(0.,0.,1.));
#26577=DIRECTION('ref_axis',(1.,0.,0.));
#26578=DIRECTION('center_axis',(0.,0.,1.));
#26579=DIRECTION('ref_axis',(1.,0.,0.));
#26580=DIRECTION('',(0.,0.,-1.));
#26581=DIRECTION('center_axis',(0.,0.,-1.));
#26582=DIRECTION('ref_axis',(-1.,0.,0.));
#26583=DIRECTION('center_axis',(0.,0.,1.));
#26584=DIRECTION('ref_axis',(1.,0.,0.));
#26585=DIRECTION('center_axis',(0.,0.,1.));
#26586=DIRECTION('ref_axis',(1.,0.,0.));
#26587=DIRECTION('center_axis',(0.,0.,1.));
#26588=DIRECTION('ref_axis',(1.,0.,0.));
#26589=DIRECTION('',(0.707106781186543,8.65956056235488E-17,-0.707106781186552));
#26590=DIRECTION('center_axis',(0.,0.,1.));
#26591=DIRECTION('ref_axis',(1.,0.,0.));
#26592=DIRECTION('center_axis',(0.,0.,1.));
#26593=DIRECTION('ref_axis',(1.,0.,0.));
#26594=DIRECTION('',(0.,0.,-1.));
#26595=DIRECTION('center_axis',(0.,0.,1.));
#26596=DIRECTION('ref_axis',(1.,0.,0.));
#26597=DIRECTION('center_axis',(0.,0.,1.));
#26598=DIRECTION('ref_axis',(1.,0.,0.));
#26599=DIRECTION('center_axis',(0.,0.,1.));
#26600=DIRECTION('ref_axis',(1.,0.,0.));
#26601=DIRECTION('center_axis',(0.,0.,1.));
#26602=DIRECTION('ref_axis',(1.,0.,0.));
#26603=DIRECTION('',(0.,0.,-1.));
#26604=DIRECTION('center_axis',(0.,0.,-1.));
#26605=DIRECTION('ref_axis',(-1.,0.,0.));
#26606=DIRECTION('center_axis',(0.,0.,1.));
#26607=DIRECTION('ref_axis',(1.,0.,0.));
#26608=DIRECTION('center_axis',(0.,0.,1.));
#26609=DIRECTION('ref_axis',(1.,0.,0.));
#26610=DIRECTION('center_axis',(0.,0.,1.));
#26611=DIRECTION('ref_axis',(1.,0.,0.));
#26612=DIRECTION('',(0.,0.,-1.));
#26613=DIRECTION('center_axis',(0.,0.,1.));
#26614=DIRECTION('ref_axis',(1.,0.,0.));
#26615=DIRECTION('center_axis',(0.,0.,1.));
#26616=DIRECTION('ref_axis',(1.,0.,0.));
#26617=DIRECTION('center_axis',(0.,0.,1.));
#26618=DIRECTION('ref_axis',(1.,0.,0.));
#26619=DIRECTION('center_axis',(0.,0.,1.));
#26620=DIRECTION('ref_axis',(1.,0.,0.));
#26621=DIRECTION('',(0.,0.,-1.));
#26622=DIRECTION('center_axis',(0.,0.,-1.));
#26623=DIRECTION('ref_axis',(-1.,0.,0.));
#26624=DIRECTION('center_axis',(0.,0.,1.));
#26625=DIRECTION('ref_axis',(1.,0.,0.));
#26626=DIRECTION('center_axis',(0.,0.,1.));
#26627=DIRECTION('ref_axis',(1.,0.,0.));
#26628=DIRECTION('center_axis',(0.,0.,1.));
#26629=DIRECTION('ref_axis',(1.,0.,0.));
#26630=DIRECTION('',(0.,0.,-1.));
#26631=DIRECTION('center_axis',(0.,0.,-1.));
#26632=DIRECTION('ref_axis',(1.,0.,0.));
#26633=DIRECTION('center_axis',(0.,0.,1.));
#26634=DIRECTION('ref_axis',(1.,0.,0.));
#26635=DIRECTION('',(-0.707106781186546,-8.65956056235491E-17,-0.707106781186549));
#26636=DIRECTION('center_axis',(0.,0.,1.));
#26637=DIRECTION('ref_axis',(1.,0.,0.));
#41847=CARTESIAN_POINT('',(0.,0.,0.));
#41848=CARTESIAN_POINT('Origin',(0.,0.,-16.505));
#41849=CARTESIAN_POINT('',(-0.24404761904762,-2.98872135506201E-17,-16.6));
#41850=CARTESIAN_POINT('Origin',(0.,0.,-16.6));
#41851=CARTESIAN_POINT('',(-0.125,-1.53080849893419E-17,-16.4));
#41852=CARTESIAN_POINT('',(-0.1875,-2.29621274840129E-17,-16.505));
#41853=CARTESIAN_POINT('Origin',(0.,0.,-16.4));
#41854=CARTESIAN_POINT('Origin',(0.,0.,-16.4));
#41855=CARTESIAN_POINT('',(0.,0.,-16.325));
#41856=CARTESIAN_POINT('',(-0.125,-1.53080849893419E-17,-16.4));
#41857=CARTESIAN_POINT('Origin',(0.75,-0.3,-14.));
#41858=CARTESIAN_POINT('',(1.05830052442584,-0.3,-15.9));
#41859=CARTESIAN_POINT('',(1.05830052442584,-0.3,-14.));
#41860=CARTESIAN_POINT('',(1.05830052442584,-0.3,-14.75));
#41861=CARTESIAN_POINT('',(0.75,-0.3,-15.9));
#41862=CARTESIAN_POINT('',(0.75,-0.3,-15.9));
#41863=CARTESIAN_POINT('',(0.75,-0.3,-14.));
#41864=CARTESIAN_POINT('',(0.75,-0.3,-15.9));
#41865=CARTESIAN_POINT('',(0.75,-0.3,-14.));
#41866=CARTESIAN_POINT('Origin',(0.75,0.,-14.));
#41867=CARTESIAN_POINT('',(1.05830052442584,0.3,-14.));
#41868=CARTESIAN_POINT('Ctrl Pts',(1.05830052442584,-0.3,-14.));
#41869=CARTESIAN_POINT('Ctrl Pts',(1.05830052442584,-0.3,-13.9621197920773));
#41870=CARTESIAN_POINT('Ctrl Pts',(1.06054662122175,-0.292390180522678,
-13.9218545194158));
#41871=CARTESIAN_POINT('Ctrl Pts',(1.06852962982332,-0.261716593696817,
-13.8480027362622));
#41872=CARTESIAN_POINT('Ctrl Pts',(1.0741374678263,-0.238662416759524,-13.8143983480476));
#41873=CARTESIAN_POINT('Ctrl Pts',(1.0845648020257,-0.185606967199746,-13.7613428984878));
#41874=CARTESIAN_POINT('Ctrl Pts',(1.09008017269667,-0.152000388353929,
-13.7382845890765));
#41875=CARTESIAN_POINT('Ctrl Pts',(1.09784922615088,-0.07814075455321,-13.7076079715749));
#41876=CARTESIAN_POINT('Ctrl Pts',(1.1,-0.0378726187868804,-13.7));
#41877=CARTESIAN_POINT('Ctrl Pts',(1.1,0.0378726187868803,-13.7));
#41878=CARTESIAN_POINT('Ctrl Pts',(1.09784922615088,0.07814075455321,-13.7076079715749));
#41879=CARTESIAN_POINT('Ctrl Pts',(1.09008017269667,0.152000388353929,-13.7382845890765));
#41880=CARTESIAN_POINT('Ctrl Pts',(1.0845648020257,0.185606967199746,-13.7613428984878));
#41881=CARTESIAN_POINT('Ctrl Pts',(1.0741374678263,0.238662416759524,-13.8143983480476));
#41882=CARTESIAN_POINT('Ctrl Pts',(1.06852962982332,0.261716593696815,-13.8480027362621));
#41883=CARTESIAN_POINT('Ctrl Pts',(1.06054662122175,0.292390180522677,-13.9218545194158));
#41884=CARTESIAN_POINT('Ctrl Pts',(1.05830052442584,0.3,-13.9621197920773));
#41885=CARTESIAN_POINT('Ctrl Pts',(1.05830052442584,0.3,-14.));
#41886=CARTESIAN_POINT('',(0.75,0.3,-14.));
#41887=CARTESIAN_POINT('Origin',(0.75,0.,-14.));
#41888=CARTESIAN_POINT('',(0.75,0.3,-14.));
#41889=CARTESIAN_POINT('Origin',(0.75,0.3,-15.9));
#41890=CARTESIAN_POINT('',(1.05830052442584,0.3,-15.9));
#41891=CARTESIAN_POINT('',(1.05830052442584,0.3,-14.75));
#41892=CARTESIAN_POINT('',(0.75,0.3,-15.9));
#41893=CARTESIAN_POINT('',(0.75,0.3,-14.));
#41894=CARTESIAN_POINT('',(0.75,0.3,-15.9));
#41895=CARTESIAN_POINT('Origin',(0.75,0.,-15.9));
#41896=CARTESIAN_POINT('Ctrl Pts',(1.05830052442584,0.3,-15.9));
#41897=CARTESIAN_POINT('Ctrl Pts',(1.05830052442584,0.3,-15.9378802079227));
#41898=CARTESIAN_POINT('Ctrl Pts',(1.06054662122175,0.292390180522678,-15.9781454805842));
#41899=CARTESIAN_POINT('Ctrl Pts',(1.06852962982332,0.261716593696816,-16.0519972637378));
#41900=CARTESIAN_POINT('Ctrl Pts',(1.0741374678263,0.238662416759525,-16.0856016519524));
#41901=CARTESIAN_POINT('Ctrl Pts',(1.0845648020257,0.185606967199746,-16.1386571015122));
#41902=CARTESIAN_POINT('Ctrl Pts',(1.09008017269667,0.15200038835393,-16.1617154109235));
#41903=CARTESIAN_POINT('Ctrl Pts',(1.09784922615088,0.0781407545532106,
-16.1923920284251));
#41904=CARTESIAN_POINT('Ctrl Pts',(1.1,0.0378726187868802,-16.2));
#41905=CARTESIAN_POINT('Ctrl Pts',(1.1,-0.0378726187868802,-16.2));
#41906=CARTESIAN_POINT('Ctrl Pts',(1.09784922615088,-0.0781407545532106,
-16.1923920284251));
#41907=CARTESIAN_POINT('Ctrl Pts',(1.09008017269667,-0.152000388353928,
-16.1617154109235));
#41908=CARTESIAN_POINT('Ctrl Pts',(1.0845648020257,-0.185606967199746,-16.1386571015122));
#41909=CARTESIAN_POINT('Ctrl Pts',(1.0741374678263,-0.238662416759525,-16.0856016519524));
#41910=CARTESIAN_POINT('Ctrl Pts',(1.06852962982332,-0.261716593696816,
-16.0519972637378));
#41911=CARTESIAN_POINT('Ctrl Pts',(1.06054662122175,-0.292390180522678,
-15.9781454805842));
#41912=CARTESIAN_POINT('Ctrl Pts',(1.05830052442584,-0.3,-15.9378802079227));
#41913=CARTESIAN_POINT('Ctrl Pts',(1.05830052442584,-0.3,-15.9));
#41914=CARTESIAN_POINT('Origin',(0.75,0.,-15.9));
#41915=CARTESIAN_POINT('Origin',(0.75,0.,-14.95));
#41916=CARTESIAN_POINT('Origin',(0.85,-0.4,-0.6));
#41917=CARTESIAN_POINT('',(1.1842719282327,-0.4,-1.4));
#41918=CARTESIAN_POINT('',(1.1842719282327,-0.4,-0.6));
#41919=CARTESIAN_POINT('',(1.1842719282327,-0.4,-3.5525));
#41920=CARTESIAN_POINT('',(0.85,-0.4,-1.4));
#41921=CARTESIAN_POINT('',(0.85,-0.4,-1.4));
#41922=CARTESIAN_POINT('',(0.85,-0.4,-0.6));
#41923=CARTESIAN_POINT('',(0.85,-0.4,-1.4));
#41924=CARTESIAN_POINT('',(0.85,-0.4,-0.6));
#41925=CARTESIAN_POINT('Origin',(0.85,2.77555756156289E-17,-0.6));
#41926=CARTESIAN_POINT('',(1.1842719282327,0.4,-0.6));
#41927=CARTESIAN_POINT('Ctrl Pts',(1.1842719282327,-0.4,-0.6));
#41928=CARTESIAN_POINT('Ctrl Pts',(1.1842719282327,-0.4,-0.549378294110008));
#41929=CARTESIAN_POINT('Ctrl Pts',(1.18785814874083,-0.389809986586072,
-0.495648946446262));
#41930=CARTESIAN_POINT('Ctrl Pts',(1.20051612521885,-0.34888367623215,-0.39721643728222));
#41931=CARTESIAN_POINT('Ctrl Pts',(1.20937438602785,-0.318164321482014,
-0.352478896532776));
#41932=CARTESIAN_POINT('Ctrl Pts',(1.22578154244013,-0.247534895635844,
-0.281849470686606));
#41933=CARTESIAN_POINT('Ctrl Pts',(1.23443746535443,-0.202791815317204,
-0.251119471874504));
#41934=CARTESIAN_POINT('Ctrl Pts',(1.24662494888297,-0.10433893315722,-0.210185257163551));
#41935=CARTESIAN_POINT('Ctrl Pts',(1.25,-0.0506019394319205,-0.2));
#41936=CARTESIAN_POINT('Ctrl Pts',(1.25,0.0506019394319202,-0.2));
#41937=CARTESIAN_POINT('Ctrl Pts',(1.24662494888297,0.10433893315722,-0.210185257163551));
#41938=CARTESIAN_POINT('Ctrl Pts',(1.23443746535443,0.202791815317204,-0.251119471874504));
#41939=CARTESIAN_POINT('Ctrl Pts',(1.22578154244013,0.247534895635844,-0.281849470686606));
#41940=CARTESIAN_POINT('Ctrl Pts',(1.20937438602785,0.318164321482014,-0.352478896532776));
#41941=CARTESIAN_POINT('Ctrl Pts',(1.20051612521885,0.34888367623215,-0.39721643728222));
#41942=CARTESIAN_POINT('Ctrl Pts',(1.18785814874083,0.389809986586072,-0.495648946446262));
#41943=CARTESIAN_POINT('Ctrl Pts',(1.1842719282327,0.4,-0.549378294110007));
#41944=CARTESIAN_POINT('Ctrl Pts',(1.1842719282327,0.4,-0.6));
#41945=CARTESIAN_POINT('',(0.85,0.4,-0.6));
#41946=CARTESIAN_POINT('Origin',(0.85,2.77555756156289E-17,-0.6));
#41947=CARTESIAN_POINT('',(0.85,0.4,-0.6));
#41948=CARTESIAN_POINT('Origin',(0.85,0.4,-1.4));
#41949=CARTESIAN_POINT('',(1.1842719282327,0.4,-1.4));
#41950=CARTESIAN_POINT('',(1.1842719282327,0.4,-3.5525));
#41951=CARTESIAN_POINT('',(0.85,0.4,-1.4));
#41952=CARTESIAN_POINT('',(0.85,0.4,-0.6));
#41953=CARTESIAN_POINT('',(0.85,0.4,-1.4));
#41954=CARTESIAN_POINT('Origin',(0.85,2.77555756156289E-17,-1.4));
#41955=CARTESIAN_POINT('Ctrl Pts',(1.1842719282327,0.4,-1.4));
#41956=CARTESIAN_POINT('Ctrl Pts',(1.1842719282327,0.4,-1.45062170588999));
#41957=CARTESIAN_POINT('Ctrl Pts',(1.18785814874083,0.389809986586072,-1.50435105355374));
#41958=CARTESIAN_POINT('Ctrl Pts',(1.20051612521885,0.34888367623215,-1.60278356271778));
#41959=CARTESIAN_POINT('Ctrl Pts',(1.20937438602785,0.318164321482014,-1.64752110346722));
#41960=CARTESIAN_POINT('Ctrl Pts',(1.22578154244013,0.247534895635844,-1.71815052931339));
#41961=CARTESIAN_POINT('Ctrl Pts',(1.23443746535443,0.202791815317204,-1.7488805281255));
#41962=CARTESIAN_POINT('Ctrl Pts',(1.24662494888297,0.10433893315722,-1.78981474283645));
#41963=CARTESIAN_POINT('Ctrl Pts',(1.25,0.0506019394319202,-1.8));
#41964=CARTESIAN_POINT('Ctrl Pts',(1.25,-0.0506019394319203,-1.8));
#41965=CARTESIAN_POINT('Ctrl Pts',(1.24662494888297,-0.10433893315722,-1.78981474283645));
#41966=CARTESIAN_POINT('Ctrl Pts',(1.23443746535443,-0.202791815317204,
-1.7488805281255));
#41967=CARTESIAN_POINT('Ctrl Pts',(1.22578154244013,-0.247534895635844,
-1.71815052931339));
#41968=CARTESIAN_POINT('Ctrl Pts',(1.20937438602785,-0.318164321482014,
-1.64752110346722));
#41969=CARTESIAN_POINT('Ctrl Pts',(1.20051612521885,-0.34888367623215,-1.60278356271778));
#41970=CARTESIAN_POINT('Ctrl Pts',(1.18785814874083,-0.389809986586072,
-1.50435105355374));
#41971=CARTESIAN_POINT('Ctrl Pts',(1.1842719282327,-0.4,-1.45062170588999));
#41972=CARTESIAN_POINT('Ctrl Pts',(1.1842719282327,-0.4,-1.4));
#41973=CARTESIAN_POINT('Origin',(0.85,2.77555756156289E-17,-1.4));
#41974=CARTESIAN_POINT('Origin',(0.85,0.,-1.));
#41975=CARTESIAN_POINT('Origin',(1.,0.,-16.6));
#41976=CARTESIAN_POINT('',(-1.,-1.22464679914736E-16,-16.6));
#41977=CARTESIAN_POINT('Origin',(0.,0.,-16.6));
#41978=CARTESIAN_POINT('Origin',(0.,0.,-16.55));
#41979=CARTESIAN_POINT('',(-1.1,-1.34711147906209E-16,-16.5));
#41980=CARTESIAN_POINT('Origin',(0.,0.,-16.5));
#41981=CARTESIAN_POINT('',(-1.05,-1.28587913910472E-16,-16.55));
#41982=CARTESIAN_POINT('Origin',(0.,0.,-14.75));
#41983=CARTESIAN_POINT('',(-1.1,-1.34711147906209E-16,-13.));
#41984=CARTESIAN_POINT('Origin',(0.,0.,-13.));
#41985=CARTESIAN_POINT('',(-1.1,-1.34711147906209E-16,-14.75));
#41986=CARTESIAN_POINT('Origin',(1.2,0.,-13.));
#41987=CARTESIAN_POINT('',(-1.2,-1.46957615897682E-16,-13.));
#41988=CARTESIAN_POINT('Origin',(0.,0.,-13.));
#41989=CARTESIAN_POINT('Origin',(0.,0.,-12.975));
#41990=CARTESIAN_POINT('',(-1.25,-1.53080849893419E-16,-12.95));
#41991=CARTESIAN_POINT('Origin',(0.,0.,-12.95));
#41992=CARTESIAN_POINT('',(-1.225,-1.50019232895551E-16,-12.975));
#41993=CARTESIAN_POINT('Origin',(0.,0.,-12.1575));
#41994=CARTESIAN_POINT('',(-1.25,-1.53080849893419E-16,-11.365));
#41995=CARTESIAN_POINT('Origin',(0.,0.,-11.365));
#41996=CARTESIAN_POINT('',(-1.25,-1.53080849893419E-16,-12.1575));
#41997=CARTESIAN_POINT('Origin',(1.195,0.,-11.365));
#41998=CARTESIAN_POINT('',(-1.195,-1.46345292498109E-16,-11.365));
#41999=CARTESIAN_POINT('Origin',(0.,0.,-11.365));
#42000=CARTESIAN_POINT('Origin',(0.,0.,-11.3));
#42001=CARTESIAN_POINT('',(-1.195,-1.46345292498109E-16,-11.235));
#42002=CARTESIAN_POINT('Origin',(0.,0.,-11.235));
#42003=CARTESIAN_POINT('',(-1.195,-1.46345292498109E-16,-11.3));
#42004=CARTESIAN_POINT('Origin',(1.25,0.,-11.235));
#42005=CARTESIAN_POINT('',(-1.25,-1.53080849893419E-16,-11.235));
#42006=CARTESIAN_POINT('Origin',(0.,0.,-11.235));
#42007=CARTESIAN_POINT('Origin',(0.,0.,-3.5525));
#42008=CARTESIAN_POINT('',(-1.25,-1.53080849893419E-16,4.13));
#42009=CARTESIAN_POINT('Origin',(0.,0.,4.13));
#42010=CARTESIAN_POINT('',(-1.25,-1.53080849893419E-16,-3.5525));
#42011=CARTESIAN_POINT('Origin',(1.195,0.,4.13));
#42012=CARTESIAN_POINT('',(-1.195,-1.46345292498109E-16,4.13));
#42013=CARTESIAN_POINT('Origin',(0.,0.,4.13));
#42014=CARTESIAN_POINT('Origin',(0.,0.,4.195));
#42015=CARTESIAN_POINT('',(-1.195,-1.46345292498109E-16,4.26));
#42016=CARTESIAN_POINT('Origin',(0.,0.,4.26));
#42017=CARTESIAN_POINT('',(-1.195,-1.46345292498109E-16,4.195));
#42018=CARTESIAN_POINT('Origin',(1.25,0.,4.26));
#42019=CARTESIAN_POINT('',(-1.25,-1.53080849893419E-16,4.26));
#42020=CARTESIAN_POINT('Origin',(0.,0.,4.26));
#42021=CARTESIAN_POINT('Origin',(0.,0.,4.28));
#42022=CARTESIAN_POINT('',(-1.25,-1.53080849893419E-16,4.3));
#42023=CARTESIAN_POINT('Origin',(0.,0.,4.3));
#42024=CARTESIAN_POINT('',(-1.25,-1.53080849893419E-16,4.28));
#42025=CARTESIAN_POINT('Origin',(0.,0.,4.35));
#42026=CARTESIAN_POINT('',(-1.15,-1.40834381901946E-16,4.4));
#42027=CARTESIAN_POINT('Origin',(0.,0.,4.4));
#42028=CARTESIAN_POINT('',(-1.2,-1.46957615897682E-16,4.35));
#42029=CARTESIAN_POINT('Origin',(0.,0.,4.4));
#59170=UNCERTAINTY_MEASURE_WITH_UNIT(LENGTH_MEASURE(0.001),#59205,
'DISTANCE_ACCURACY_VALUE',
'Maximum model space distance between geometric entities at asserted c
onnectivities');
#59182=UNCERTAINTY_MEASURE_WITH_UNIT(LENGTH_MEASURE(0.001),#59205,
'DISTANCE_ACCURACY_VALUE',
'Maximum model space distance between geometric entities at asserted c
onnectivities');
#59192=(
GEOMETRIC_REPRESENTATION_CONTEXT(3)
GLOBAL_UNCERTAINTY_ASSIGNED_CONTEXT((#59170))
GLOBAL_UNIT_ASSIGNED_CONTEXT((#59205,#59207,#59208))
REPRESENTATION_CONTEXT('','3D')
);
#59204=(
GEOMETRIC_REPRESENTATION_CONTEXT(3)
GLOBAL_UNCERTAINTY_ASSIGNED_CONTEXT((#59182))
GLOBAL_UNIT_ASSIGNED_CONTEXT((#59205,#59207,#59208))
REPRESENTATION_CONTEXT('','3D')
);
#59205=(
LENGTH_UNIT()
NAMED_UNIT(*)
SI_UNIT(.CENTI.,.METRE.)
);
#59207=(
NAMED_UNIT(*)
PLANE_ANGLE_UNIT()
SI_UNIT($,.RADIAN.)
);
#59208=(
NAMED_UNIT(*)
SI_UNIT($,.STERADIAN.)
SOLID_ANGLE_UNIT()
);
#59218=SHAPE_DEFINITION_REPRESENTATION(#59239,#59305);
#59239=PRODUCT_DEFINITION_SHAPE('',$,#59327);
#59305=SHAPE_REPRESENTATION('',(#23559),#59192);
#59317=PRODUCT_DEFINITION_CONTEXT('part definition',#59382,'design');
#59327=PRODUCT_DEFINITION('2026-10-23-00-47-53-406',
'04_Drive_Shaft_D25_Keyed_42CrMo4',#59348,#59317);
#59348=PRODUCT_DEFINITION_FORMATION('',$,#59393);
#59382=APPLICATION_CONTEXT(
'Core Data for Automotive Mechanical Design Process');
#59383=PRODUCT_CONTEXT('part definition',#59382,'mechanical');
#59393=PRODUCT('2026-10-23-00-47-53-406',
'04_Drive_Shaft_D25_Keyed_42CrMo4',$,(#59383));
#59580=COLOUR_RGB('Grey',0.48,0.52,0.57);
#59581=FILL_AREA_STYLE_COLOUR('',#59580);
#59582=FILL_AREA_STYLE('',(#59581));
#59583=SURFACE_STYLE_FILL_AREA(#59582);
#59584=SURFACE_SIDE_STYLE('',(#59583));
#59585=SURFACE_STYLE_USAGE(.BOTH.,#59584);
#59586=PRESENTATION_STYLE_ASSIGNMENT((#59585));
ENDSEC;
END-ISO-10303-21;
